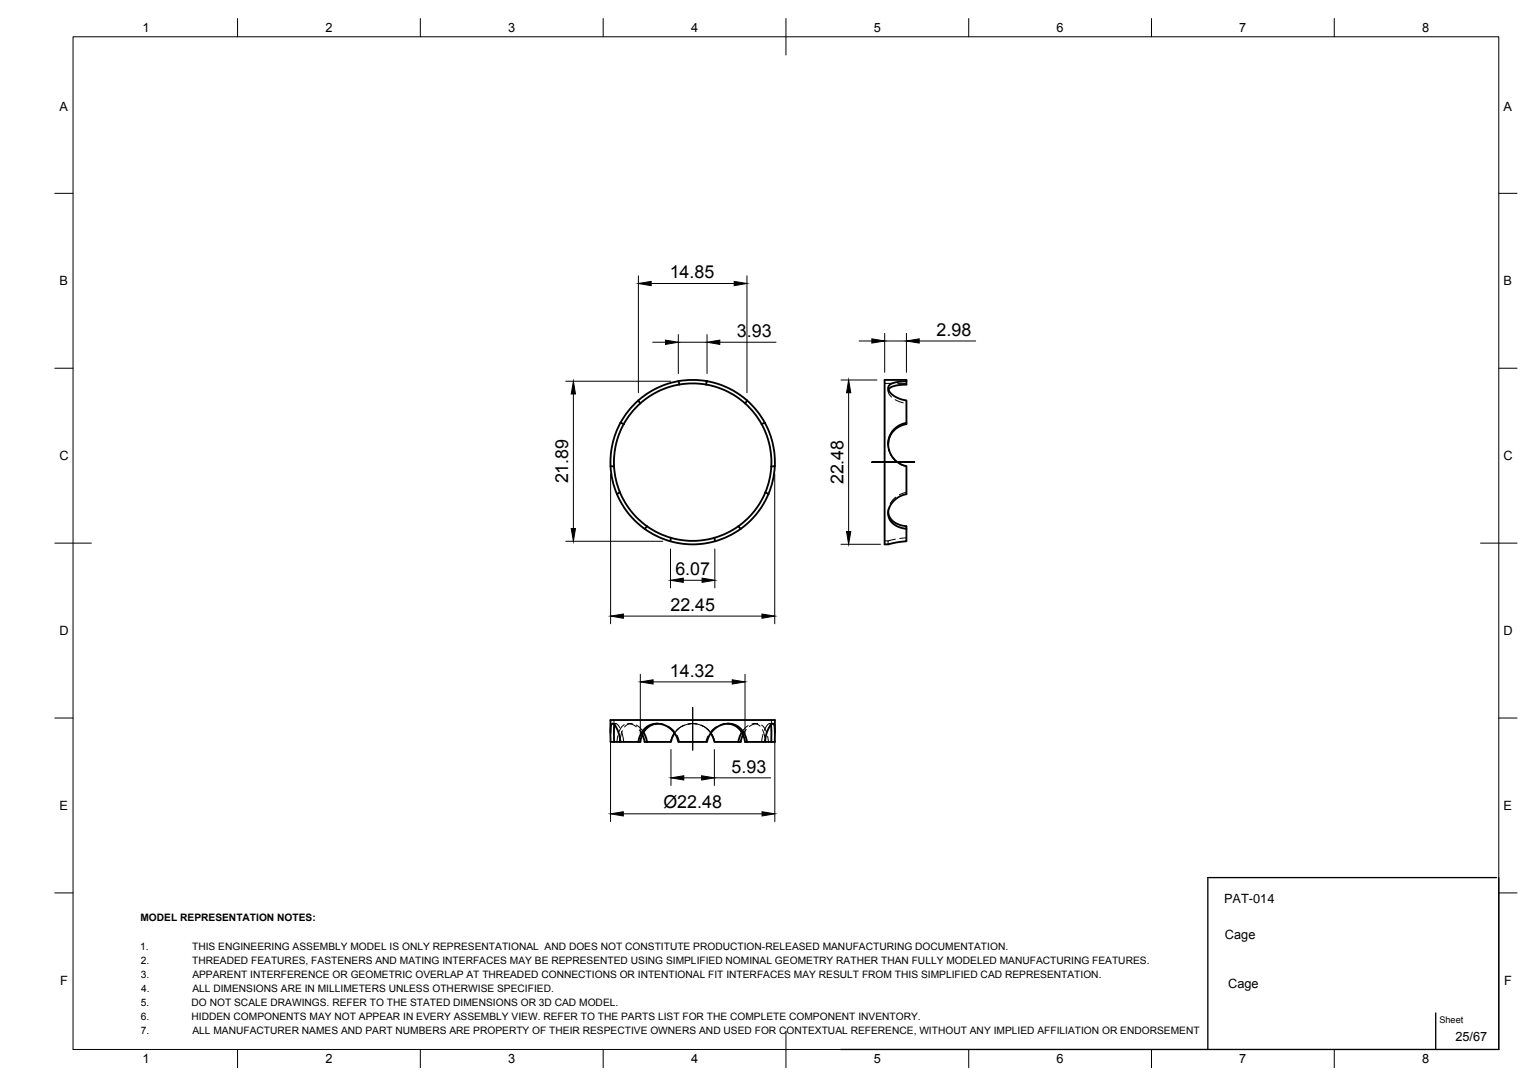
ISO-10303-21;
HEADER;
/* Generated by software containing ST-Developer
 * from STEP Tools, Inc. (www.steptools.com) 
 */

FILE_DESCRIPTION(
/* description */ ('Bin tilter linkage'),
/* implementation_level */ '2;1');

FILE_NAME(
/* name */ 'Cage.step',
/* time_stamp */ '2026-10-28T03:26:24-07:00',
/* author */ (''),
/* organization */ (''),
/* preprocessor_version */ 'ST-DEVELOPER v20.2',
/* originating_system */ 'Autodesk Translation Framework v15.17.0.0',
/* authorisation */ '');

FILE_SCHEMA (('AUTOMOTIVE_DESIGN { 1 0 10303 214 3 1 1 }'));
ENDSEC;

DATA;
#10=MECHANICAL_DESIGN_GEOMETRIC_PRESENTATION_REPRESENTATION('',(#943),#23728);
#599=B_SPLINE_CURVE_WITH_KNOTS('',3,(#21962,#21963,#21964,#21965,#21966,
#21967,#21968,#21969,#21970,#21971,#21972,#21973,#21974,#21975,#21976,#21977,
#21978,#21979,#21980,#21981,#21982,#21983),.UNSPECIFIED.,.F.,.F.,(4,2,2,
2,2,2,2,2,2,2,4),(0.0591825211272536,0.157966726598481,0.236950089897721,
0.315933453196962,0.391576304923761,0.46721915665056,0.54286200837736,0.618504860104159,
0.697488223403399,0.77647158670264,0.875255792173867),.UNSPECIFIED.);
#600=B_SPLINE_CURVE_WITH_KNOTS('',3,(#21987,#21988,#21989,#21990,#21991,
#21992,#21993,#21994,#21995,#21996,#21997,#21998,#21999,#22000,#22001,#22002,
#22003,#22004,#22005,#22006,#22007,#22008),.UNSPECIFIED.,.F.,.F.,(4,2,2,
2,2,2,2,2,2,2,4),(0.0581119756758434,0.106553146291161,0.213106292582322,
0.30849933801665,0.386091982889075,0.4636846277615,0.541277272633925,0.61886991750635,
0.714262962940678,0.820816109231839,0.869257279847157),.UNSPECIFIED.);
#601=B_SPLINE_CURVE_WITH_KNOTS('',3,(#22014,#22015,#22016,#22017,#22018,
#22019,#22020,#22021,#22022,#22023,#22024,#22025,#22026,#22027,#22028,#22029,
#22030,#22031,#22032,#22033,#22034,#22035),.UNSPECIFIED.,.F.,.F.,(4,2,2,
2,2,2,2,2,2,2,4),(0.0581119756758434,0.106553146291161,0.213106292582322,
0.30849933801665,0.386091982889075,0.4636846277615,0.541277272633925,0.61886991750635,
0.714262962940679,0.820816109231839,0.869257279847157),.UNSPECIFIED.);
#602=B_SPLINE_CURVE_WITH_KNOTS('',3,(#22039,#22040,#22041,#22042,#22043,
#22044,#22045,#22046,#22047,#22048,#22049,#22050,#22051,#22052,#22053,#22054,
#22055,#22056,#22057,#22058,#22059,#22060),.UNSPECIFIED.,.F.,.F.,(4,2,2,
2,2,2,2,2,2,2,4),(0.0581119756758433,0.106553146291161,0.213106292582322,
0.308499338016649,0.386091982889075,0.4636846277615,0.541277272633925,0.61886991750635,
0.714262962940678,0.820816109231839,0.869257279847157),.UNSPECIFIED.);
#603=B_SPLINE_CURVE_WITH_KNOTS('',3,(#22069,#22070,#22071,#22072,#22073,
#22074,#22075,#22076,#22077,#22078,#22079,#22080,#22081,#22082,#22083,#22084,
#22085,#22086,#22087,#22088,#22089,#22090),.UNSPECIFIED.,.F.,.F.,(4,2,2,
2,2,2,2,2,2,2,4),(0.0581119756758433,0.106553146291161,0.213106292582322,
0.30849933801665,0.386091982889075,0.4636846277615,0.541277272633925,0.61886991750635,
0.714262962940678,0.820816109231839,0.869257279847157),.UNSPECIFIED.);
#604=B_SPLINE_CURVE_WITH_KNOTS('',3,(#22094,#22095,#22096,#22097,#22098,
#22099,#22100,#22101,#22102,#22103,#22104,#22105,#22106,#22107,#22108,#22109,
#22110,#22111,#22112,#22113,#22114,#22115),.UNSPECIFIED.,.F.,.F.,(4,2,2,
2,2,2,2,2,2,2,4),(0.0581119756758434,0.106553146291161,0.213106292582322,
0.30849933801665,0.386091982889075,0.4636846277615,0.541277272633925,0.61886991750635,
0.714262962940678,0.820816109231839,0.869257279847157),.UNSPECIFIED.);
#605=B_SPLINE_CURVE_WITH_KNOTS('',3,(#22119,#22120,#22121,#22122,#22123,
#22124,#22125,#22126,#22127,#22128,#22129,#22130,#22131,#22132,#22133,#22134,
#22135,#22136,#22137,#22138,#22139,#22140),.UNSPECIFIED.,.F.,.F.,(4,2,2,
2,2,2,2,2,2,2,4),(0.0581119756758434,0.106553146291161,0.213106292582322,
0.30849933801665,0.386091982889075,0.4636846277615,0.541277272633925,0.61886991750635,
0.714262962940678,0.820816109231839,0.869257279847157),.UNSPECIFIED.);
#606=B_SPLINE_CURVE_WITH_KNOTS('',3,(#22144,#22145,#22146,#22147,#22148,
#22149,#22150,#22151,#22152,#22153,#22154,#22155,#22156,#22157,#22158,#22159,
#22160,#22161,#22162,#22163,#22164,#22165),.UNSPECIFIED.,.F.,.F.,(4,2,2,
2,2,2,2,2,2,2,4),(0.0581119756758433,0.106553146291161,0.213106292582322,
0.30849933801665,0.386091982889075,0.4636846277615,0.541277272633925,0.61886991750635,
0.714262962940678,0.820816109231839,0.869257279847157),.UNSPECIFIED.);
#607=B_SPLINE_CURVE_WITH_KNOTS('',3,(#22173,#22174,#22175,#22176,#22177,
#22178,#22179,#22180,#22181,#22182,#22183,#22184,#22185,#22186,#22187,#22188,
#22189,#22190,#22191,#22192,#22193,#22194),.UNSPECIFIED.,.F.,.F.,(4,2,2,
2,2,2,2,2,2,2,4),(0.0591825211272536,0.157966726598481,0.236950089897721,
0.315933453196962,0.391576304923761,0.467219156650561,0.54286200837736,
0.618504860104159,0.697488223403399,0.77647158670264,0.875255792173867),
 .UNSPECIFIED.);
#608=B_SPLINE_CURVE_WITH_KNOTS('',3,(#22202,#22203,#22204,#22205,#22206,
#22207,#22208,#22209,#22210,#22211,#22212,#22213,#22214,#22215,#22216,#22217,
#22218,#22219,#22220,#22221,#22222,#22223),.UNSPECIFIED.,.F.,.F.,(4,2,2,
2,2,2,2,2,2,2,4),(0.0591825211272536,0.157966726598481,0.236950089897722,
0.315933453196962,0.391576304923761,0.467219156650561,0.54286200837736,
0.618504860104159,0.697488223403399,0.77647158670264,0.875255792173867),
 .UNSPECIFIED.);
#609=B_SPLINE_CURVE_WITH_KNOTS('',3,(#22233,#22234,#22235,#22236,#22237,
#22238,#22239,#22240,#22241,#22242,#22243,#22244,#22245,#22246,#22247,#22248,
#22249,#22250,#22251,#22252,#22253,#22254),.UNSPECIFIED.,.F.,.F.,(4,2,2,
2,2,2,2,2,2,2,4),(0.0591825211272536,0.157966726598481,0.236950089897721,
0.315933453196962,0.391576304923761,0.46721915665056,0.54286200837736,0.618504860104159,
0.697488223403399,0.77647158670264,0.875255792173867),.UNSPECIFIED.);
#610=B_SPLINE_CURVE_WITH_KNOTS('',3,(#22262,#22263,#22264,#22265,#22266,
#22267,#22268,#22269,#22270,#22271,#22272,#22273,#22274,#22275,#22276,#22277,
#22278,#22279,#22280,#22281,#22282,#22283),.UNSPECIFIED.,.F.,.F.,(4,2,2,
2,2,2,2,2,2,2,4),(0.0591825211272536,0.157966726598481,0.236950089897721,
0.315933453196962,0.391576304923761,0.46721915665056,0.542862008377359,
0.618504860104159,0.697488223403399,0.776471586702639,0.875255792173867),
 .UNSPECIFIED.);
#611=B_SPLINE_CURVE_WITH_KNOTS('',3,(#22291,#22292,#22293,#22294,#22295,
#22296,#22297,#22298,#22299,#22300,#22301,#22302,#22303,#22304,#22305,#22306,
#22307,#22308,#22309,#22310,#22311,#22312),.UNSPECIFIED.,.F.,.F.,(4,2,2,
2,2,2,2,2,2,2,4),(0.0591825211272536,0.157966726598481,0.236950089897721,
0.315933453196962,0.391576304923761,0.46721915665056,0.54286200837736,0.618504860104159,
0.697488223403399,0.77647158670264,0.875255792173867),.UNSPECIFIED.);
#612=B_SPLINE_CURVE_WITH_KNOTS('',3,(#22321,#22322,#22323,#22324,#22325,
#22326,#22327,#22328,#22329,#22330,#22331,#22332,#22333,#22334,#22335,#22336,
#22337,#22338,#22339,#22340,#22341,#22342),.UNSPECIFIED.,.F.,.F.,(4,2,2,
2,2,2,2,2,2,2,4),(0.0591825211272536,0.157966726598481,0.236950089897721,
0.315933453196962,0.391576304923761,0.46721915665056,0.542862008377359,
0.618504860104159,0.697488223403399,0.776471586702639,0.875255792173867),
 .UNSPECIFIED.);
#620=SPHERICAL_SURFACE('',#14830,0.309556);
#621=SPHERICAL_SURFACE('',#14846,0.309556);
#622=SPHERICAL_SURFACE('',#14851,0.309556);
#623=SPHERICAL_SURFACE('',#14857,0.309556);
#624=SPHERICAL_SURFACE('',#14862,0.309556);
#625=SPHERICAL_SURFACE('',#14867,0.309556);
#626=SPHERICAL_SURFACE('',#14875,0.309556);
#725=SHAPE_REPRESENTATION_RELATIONSHIP('SRR','None',#24192,#831);
#831=ADVANCED_BREP_SHAPE_REPRESENTATION('',(#1056),#23692);
#943=STYLED_ITEM('',(#24765),#1056);
#1056=MANIFOLD_SOLID_BREP('Continuous crown cage',#12474);
#1390=FACE_BOUND('',#3514,.T.);
#1741=PLANE('',#14843);
#1742=PLANE('',#14848);
#1743=PLANE('',#14853);
#1744=PLANE('',#14859);
#1745=PLANE('',#14864);
#1746=PLANE('',#14873);
#1747=PLANE('',#14877);
#1748=PLANE('',#14878);
#2418=FACE_OUTER_BOUND('',#3498,.T.);
#2419=FACE_OUTER_BOUND('',#3499,.T.);
#2420=FACE_OUTER_BOUND('',#3500,.T.);
#2421=FACE_OUTER_BOUND('',#3501,.T.);
#2422=FACE_OUTER_BOUND('',#3502,.T.);
#2423=FACE_OUTER_BOUND('',#3503,.T.);
#2424=FACE_OUTER_BOUND('',#3504,.T.);
#2425=FACE_OUTER_BOUND('',#3505,.T.);
#2426=FACE_OUTER_BOUND('',#3506,.T.);
#2427=FACE_OUTER_BOUND('',#3507,.T.);
#2428=FACE_OUTER_BOUND('',#3508,.T.);
#2429=FACE_OUTER_BOUND('',#3509,.T.);
#2430=FACE_OUTER_BOUND('',#3510,.T.);
#2431=FACE_OUTER_BOUND('',#3511,.T.);
#2432=FACE_OUTER_BOUND('',#3512,.T.);
#2433=FACE_OUTER_BOUND('',#3513,.T.);
#2434=FACE_OUTER_BOUND('',#3515,.T.);
#3498=EDGE_LOOP('',(#10291,#10292,#10293,#10294));
#3499=EDGE_LOOP('',(#10295,#10296,#10297,#10298,#10299,#10300,#10301,#10302,
#10303,#10304,#10305,#10306,#10307,#10308,#10309,#10310,#10311,#10312));
#3500=EDGE_LOOP('',(#10313,#10314,#10315,#10316));
#3501=EDGE_LOOP('',(#10317,#10318,#10319,#10320));
#3502=EDGE_LOOP('',(#10321,#10322,#10323,#10324));
#3503=EDGE_LOOP('',(#10325,#10326,#10327,#10328));
#3504=EDGE_LOOP('',(#10329,#10330,#10331,#10332,#10333,#10334));
#3505=EDGE_LOOP('',(#10335,#10336,#10337,#10338));
#3506=EDGE_LOOP('',(#10339,#10340,#10341,#10342));
#3507=EDGE_LOOP('',(#10343,#10344,#10345,#10346));
#3508=EDGE_LOOP('',(#10347,#10348,#10349,#10350));
#3509=EDGE_LOOP('',(#10351,#10352,#10353,#10354));
#3510=EDGE_LOOP('',(#10355,#10356,#10357,#10358,#10359,#10360,#10361,#10362,
#10363,#10364,#10365,#10366,#10367,#10368,#10369,#10370,#10371,#10372));
#3511=EDGE_LOOP('',(#10373,#10374,#10375,#10376));
#3512=EDGE_LOOP('',(#10377,#10378,#10379,#10380));
#3513=EDGE_LOOP('',(#10381));
#3514=EDGE_LOOP('',(#10382));
#3515=EDGE_LOOP('',(#10383,#10384,#10385,#10386));
#4263=LINE('',#22064,#4938);
#4264=LINE('',#22317,#4939);
#4938=VECTOR('',#18210,1.123812);
#4939=VECTOR('',#18279,1.076188);
#5744=CIRCLE('',#14831,0.303778037777585);
#5745=CIRCLE('',#14832,0.303778037777585);
#5746=CIRCLE('',#14834,1.123812);
#5747=CIRCLE('',#14835,1.123812);
#5748=CIRCLE('',#14836,1.123812);
#5749=CIRCLE('',#14837,1.123812);
#5750=CIRCLE('',#14838,1.123812);
#5751=CIRCLE('',#14839,1.123812);
#5752=CIRCLE('',#14840,1.123812);
#5753=CIRCLE('',#14841,1.123812);
#5754=CIRCLE('',#14842,1.123812);
#5755=CIRCLE('',#14844,1.076188);
#5756=CIRCLE('',#14845,0.303778037777585);
#5757=CIRCLE('',#14847,0.303778037777585);
#5758=CIRCLE('',#14849,1.076188);
#5759=CIRCLE('',#14850,0.303778037777585);
#5760=CIRCLE('',#14852,0.303778037777585);
#5761=CIRCLE('',#14854,1.076188);
#5762=CIRCLE('',#14855,1.076188);
#5763=CIRCLE('',#14856,0.303778037777585);
#5764=CIRCLE('',#14858,0.303778037777585);
#5765=CIRCLE('',#14860,1.076188);
#5766=CIRCLE('',#14861,0.303778037777585);
#5767=CIRCLE('',#14863,0.303778037777585);
#5768=CIRCLE('',#14865,1.076188);
#5769=CIRCLE('',#14866,0.303778037777585);
#5770=CIRCLE('',#14868,0.303778037777585);
#5771=CIRCLE('',#14870,1.076188);
#5772=CIRCLE('',#14871,1.076188);
#5773=CIRCLE('',#14872,1.076188);
#5774=CIRCLE('',#14874,0.303778037777585);
#5775=CIRCLE('',#14876,0.303778037777585);
#6603=VERTEX_POINT('',#21960);
#6604=VERTEX_POINT('',#21961);
#6605=VERTEX_POINT('',#21984);
#6606=VERTEX_POINT('',#21986);
#6607=VERTEX_POINT('',#22011);
#6608=VERTEX_POINT('',#22013);
#6609=VERTEX_POINT('',#22036);
#6610=VERTEX_POINT('',#22038);
#6611=VERTEX_POINT('',#22061);
#6612=VERTEX_POINT('',#22063);
#6613=VERTEX_POINT('',#22066);
#6614=VERTEX_POINT('',#22068);
#6615=VERTEX_POINT('',#22091);
#6616=VERTEX_POINT('',#22093);
#6617=VERTEX_POINT('',#22116);
#6618=VERTEX_POINT('',#22118);
#6619=VERTEX_POINT('',#22141);
#6620=VERTEX_POINT('',#22143);
#6621=VERTEX_POINT('',#22168);
#6622=VERTEX_POINT('',#22172);
#6623=VERTEX_POINT('',#22197);
#6624=VERTEX_POINT('',#22201);
#6625=VERTEX_POINT('',#22226);
#6626=VERTEX_POINT('',#22228);
#6627=VERTEX_POINT('',#22232);
#6628=VERTEX_POINT('',#22257);
#6629=VERTEX_POINT('',#22261);
#6630=VERTEX_POINT('',#22286);
#6631=VERTEX_POINT('',#22290);
#6632=VERTEX_POINT('',#22315);
#6633=VERTEX_POINT('',#22318);
#6634=VERTEX_POINT('',#22320);
#7885=EDGE_CURVE('',#6603,#6604,#599,.T.);
#7886=EDGE_CURVE('',#6605,#6603,#5744,.T.);
#7887=EDGE_CURVE('',#6606,#6605,#600,.T.);
#7888=EDGE_CURVE('',#6604,#6606,#5745,.T.);
#7889=EDGE_CURVE('',#6607,#6605,#5746,.T.);
#7890=EDGE_CURVE('',#6607,#6608,#601,.T.);
#7891=EDGE_CURVE('',#6609,#6608,#5747,.T.);
#7892=EDGE_CURVE('',#6609,#6610,#602,.T.);
#7893=EDGE_CURVE('',#6611,#6610,#5748,.T.);
#7894=EDGE_CURVE('',#6611,#6612,#4263,.T.);
#7895=EDGE_CURVE('',#6612,#6612,#5749,.T.);
#7896=EDGE_CURVE('',#6613,#6611,#5750,.T.);
#7897=EDGE_CURVE('',#6613,#6614,#603,.T.);
#7898=EDGE_CURVE('',#6615,#6614,#5751,.T.);
#7899=EDGE_CURVE('',#6615,#6616,#604,.T.);
#7900=EDGE_CURVE('',#6617,#6616,#5752,.T.);
#7901=EDGE_CURVE('',#6617,#6618,#605,.T.);
#7902=EDGE_CURVE('',#6619,#6618,#5753,.T.);
#7903=EDGE_CURVE('',#6619,#6620,#606,.T.);
#7904=EDGE_CURVE('',#6606,#6620,#5754,.T.);
#7905=EDGE_CURVE('',#6603,#6621,#5755,.T.);
#7906=EDGE_CURVE('',#6621,#6607,#5756,.T.);
#7907=EDGE_CURVE('',#6622,#6621,#607,.T.);
#7908=EDGE_CURVE('',#6608,#6622,#5757,.T.);
#7909=EDGE_CURVE('',#6622,#6623,#5758,.T.);
#7910=EDGE_CURVE('',#6623,#6609,#5759,.T.);
#7911=EDGE_CURVE('',#6624,#6623,#608,.T.);
#7912=EDGE_CURVE('',#6610,#6624,#5760,.T.);
#7913=EDGE_CURVE('',#6624,#6625,#5761,.T.);
#7914=EDGE_CURVE('',#6625,#6626,#5762,.T.);
#7915=EDGE_CURVE('',#6626,#6613,#5763,.T.);
#7916=EDGE_CURVE('',#6627,#6626,#609,.T.);
#7917=EDGE_CURVE('',#6614,#6627,#5764,.T.);
#7918=EDGE_CURVE('',#6627,#6628,#5765,.T.);
#7919=EDGE_CURVE('',#6628,#6615,#5766,.T.);
#7920=EDGE_CURVE('',#6629,#6628,#610,.T.);
#7921=EDGE_CURVE('',#6616,#6629,#5767,.T.);
#7922=EDGE_CURVE('',#6629,#6630,#5768,.T.);
#7923=EDGE_CURVE('',#6630,#6617,#5769,.T.);
#7924=EDGE_CURVE('',#6631,#6630,#611,.T.);
#7925=EDGE_CURVE('',#6618,#6631,#5770,.T.);
#7926=EDGE_CURVE('',#6632,#6632,#5771,.T.);
#7927=EDGE_CURVE('',#6632,#6625,#4264,.T.);
#7928=EDGE_CURVE('',#6633,#6604,#5772,.T.);
#7929=EDGE_CURVE('',#6633,#6634,#612,.T.);
#7930=EDGE_CURVE('',#6631,#6634,#5773,.T.);
#7931=EDGE_CURVE('',#6620,#6633,#5774,.T.);
#7932=EDGE_CURVE('',#6634,#6619,#5775,.T.);
#10291=ORIENTED_EDGE('',*,*,#7885,.F.);
#10292=ORIENTED_EDGE('',*,*,#7886,.F.);
#10293=ORIENTED_EDGE('',*,*,#7887,.F.);
#10294=ORIENTED_EDGE('',*,*,#7888,.F.);
#10295=ORIENTED_EDGE('',*,*,#7887,.T.);
#10296=ORIENTED_EDGE('',*,*,#7889,.F.);
#10297=ORIENTED_EDGE('',*,*,#7890,.T.);
#10298=ORIENTED_EDGE('',*,*,#7891,.F.);
#10299=ORIENTED_EDGE('',*,*,#7892,.T.);
#10300=ORIENTED_EDGE('',*,*,#7893,.F.);
#10301=ORIENTED_EDGE('',*,*,#7894,.T.);
#10302=ORIENTED_EDGE('',*,*,#7895,.F.);
#10303=ORIENTED_EDGE('',*,*,#7894,.F.);
#10304=ORIENTED_EDGE('',*,*,#7896,.F.);
#10305=ORIENTED_EDGE('',*,*,#7897,.T.);
#10306=ORIENTED_EDGE('',*,*,#7898,.F.);
#10307=ORIENTED_EDGE('',*,*,#7899,.T.);
#10308=ORIENTED_EDGE('',*,*,#7900,.F.);
#10309=ORIENTED_EDGE('',*,*,#7901,.T.);
#10310=ORIENTED_EDGE('',*,*,#7902,.F.);
#10311=ORIENTED_EDGE('',*,*,#7903,.T.);
#10312=ORIENTED_EDGE('',*,*,#7904,.F.);
#10313=ORIENTED_EDGE('',*,*,#7886,.T.);
#10314=ORIENTED_EDGE('',*,*,#7905,.T.);
#10315=ORIENTED_EDGE('',*,*,#7906,.T.);
#10316=ORIENTED_EDGE('',*,*,#7889,.T.);
#10317=ORIENTED_EDGE('',*,*,#7907,.F.);
#10318=ORIENTED_EDGE('',*,*,#7908,.F.);
#10319=ORIENTED_EDGE('',*,*,#7890,.F.);
#10320=ORIENTED_EDGE('',*,*,#7906,.F.);
#10321=ORIENTED_EDGE('',*,*,#7908,.T.);
#10322=ORIENTED_EDGE('',*,*,#7909,.T.);
#10323=ORIENTED_EDGE('',*,*,#7910,.T.);
#10324=ORIENTED_EDGE('',*,*,#7891,.T.);
#10325=ORIENTED_EDGE('',*,*,#7911,.F.);
#10326=ORIENTED_EDGE('',*,*,#7912,.F.);
#10327=ORIENTED_EDGE('',*,*,#7892,.F.);
#10328=ORIENTED_EDGE('',*,*,#7910,.F.);
#10329=ORIENTED_EDGE('',*,*,#7912,.T.);
#10330=ORIENTED_EDGE('',*,*,#7913,.T.);
#10331=ORIENTED_EDGE('',*,*,#7914,.T.);
#10332=ORIENTED_EDGE('',*,*,#7915,.T.);
#10333=ORIENTED_EDGE('',*,*,#7896,.T.);
#10334=ORIENTED_EDGE('',*,*,#7893,.T.);
#10335=ORIENTED_EDGE('',*,*,#7916,.F.);
#10336=ORIENTED_EDGE('',*,*,#7917,.F.);
#10337=ORIENTED_EDGE('',*,*,#7897,.F.);
#10338=ORIENTED_EDGE('',*,*,#7915,.F.);
#10339=ORIENTED_EDGE('',*,*,#7917,.T.);
#10340=ORIENTED_EDGE('',*,*,#7918,.T.);
#10341=ORIENTED_EDGE('',*,*,#7919,.T.);
#10342=ORIENTED_EDGE('',*,*,#7898,.T.);
#10343=ORIENTED_EDGE('',*,*,#7920,.F.);
#10344=ORIENTED_EDGE('',*,*,#7921,.F.);
#10345=ORIENTED_EDGE('',*,*,#7899,.F.);
#10346=ORIENTED_EDGE('',*,*,#7919,.F.);
#10347=ORIENTED_EDGE('',*,*,#7921,.T.);
#10348=ORIENTED_EDGE('',*,*,#7922,.T.);
#10349=ORIENTED_EDGE('',*,*,#7923,.T.);
#10350=ORIENTED_EDGE('',*,*,#7900,.T.);
#10351=ORIENTED_EDGE('',*,*,#7901,.F.);
#10352=ORIENTED_EDGE('',*,*,#7923,.F.);
#10353=ORIENTED_EDGE('',*,*,#7924,.F.);
#10354=ORIENTED_EDGE('',*,*,#7925,.F.);
#10355=ORIENTED_EDGE('',*,*,#7926,.F.);
#10356=ORIENTED_EDGE('',*,*,#7927,.T.);
#10357=ORIENTED_EDGE('',*,*,#7913,.F.);
#10358=ORIENTED_EDGE('',*,*,#7911,.T.);
#10359=ORIENTED_EDGE('',*,*,#7909,.F.);
#10360=ORIENTED_EDGE('',*,*,#7907,.T.);
#10361=ORIENTED_EDGE('',*,*,#7905,.F.);
#10362=ORIENTED_EDGE('',*,*,#7885,.T.);
#10363=ORIENTED_EDGE('',*,*,#7928,.F.);
#10364=ORIENTED_EDGE('',*,*,#7929,.T.);
#10365=ORIENTED_EDGE('',*,*,#7930,.F.);
#10366=ORIENTED_EDGE('',*,*,#7924,.T.);
#10367=ORIENTED_EDGE('',*,*,#7922,.F.);
#10368=ORIENTED_EDGE('',*,*,#7920,.T.);
#10369=ORIENTED_EDGE('',*,*,#7918,.F.);
#10370=ORIENTED_EDGE('',*,*,#7916,.T.);
#10371=ORIENTED_EDGE('',*,*,#7914,.F.);
#10372=ORIENTED_EDGE('',*,*,#7927,.F.);
#10373=ORIENTED_EDGE('',*,*,#7888,.T.);
#10374=ORIENTED_EDGE('',*,*,#7904,.T.);
#10375=ORIENTED_EDGE('',*,*,#7931,.T.);
#10376=ORIENTED_EDGE('',*,*,#7928,.T.);
#10377=ORIENTED_EDGE('',*,*,#7903,.F.);
#10378=ORIENTED_EDGE('',*,*,#7932,.F.);
#10379=ORIENTED_EDGE('',*,*,#7929,.F.);
#10380=ORIENTED_EDGE('',*,*,#7931,.F.);
#10381=ORIENTED_EDGE('',*,*,#7895,.T.);
#10382=ORIENTED_EDGE('',*,*,#7926,.T.);
#10383=ORIENTED_EDGE('',*,*,#7925,.T.);
#10384=ORIENTED_EDGE('',*,*,#7930,.T.);
#10385=ORIENTED_EDGE('',*,*,#7932,.T.);
#10386=ORIENTED_EDGE('',*,*,#7902,.T.);
#11529=CYLINDRICAL_SURFACE('',#14833,1.123812);
#11530=CYLINDRICAL_SURFACE('',#14869,1.076188);
#12143=ADVANCED_FACE('',(#2418),#620,.F.);
#12144=ADVANCED_FACE('',(#2419),#11529,.T.);
#12145=ADVANCED_FACE('',(#2420),#1741,.T.);
#12146=ADVANCED_FACE('',(#2421),#621,.F.);
#12147=ADVANCED_FACE('',(#2422),#1742,.T.);
#12148=ADVANCED_FACE('',(#2423),#622,.F.);
#12149=ADVANCED_FACE('',(#2424),#1743,.T.);
#12150=ADVANCED_FACE('',(#2425),#623,.F.);
#12151=ADVANCED_FACE('',(#2426),#1744,.T.);
#12152=ADVANCED_FACE('',(#2427),#624,.F.);
#12153=ADVANCED_FACE('',(#2428),#1745,.T.);
#12154=ADVANCED_FACE('',(#2429),#625,.F.);
#12155=ADVANCED_FACE('',(#2430),#11530,.F.);
#12156=ADVANCED_FACE('',(#2431),#1746,.T.);
#12157=ADVANCED_FACE('',(#2432),#626,.F.);
#12158=ADVANCED_FACE('',(#2433,#1390),#1747,.T.);
#12159=ADVANCED_FACE('',(#2434),#1748,.T.);
#12474=CLOSED_SHELL('',(#12143,#12144,#12145,#12146,#12147,#12148,#12149,
#12150,#12151,#12152,#12153,#12154,#12155,#12156,#12157,#12158,#12159));
#14829=AXIS2_PLACEMENT_3D('',#21958,#18194,#18195);
#14830=AXIS2_PLACEMENT_3D('',#21959,#18196,#18197);
#14831=AXIS2_PLACEMENT_3D('',#21985,#18198,#18199);
#14832=AXIS2_PLACEMENT_3D('',#22009,#18200,#18201);
#14833=AXIS2_PLACEMENT_3D('',#22010,#18202,#18203);
#14834=AXIS2_PLACEMENT_3D('',#22012,#18204,#18205);
#14835=AXIS2_PLACEMENT_3D('',#22037,#18206,#18207);
#14836=AXIS2_PLACEMENT_3D('',#22062,#18208,#18209);
#14837=AXIS2_PLACEMENT_3D('',#22065,#18211,#18212);
#14838=AXIS2_PLACEMENT_3D('',#22067,#18213,#18214);
#14839=AXIS2_PLACEMENT_3D('',#22092,#18215,#18216);
#14840=AXIS2_PLACEMENT_3D('',#22117,#18217,#18218);
#14841=AXIS2_PLACEMENT_3D('',#22142,#18219,#18220);
#14842=AXIS2_PLACEMENT_3D('',#22166,#18221,#18222);
#14843=AXIS2_PLACEMENT_3D('',#22167,#18223,#18224);
#14844=AXIS2_PLACEMENT_3D('',#22169,#18225,#18226);
#14845=AXIS2_PLACEMENT_3D('',#22170,#18227,#18228);
#14846=AXIS2_PLACEMENT_3D('',#22171,#18229,#18230);
#14847=AXIS2_PLACEMENT_3D('',#22195,#18231,#18232);
#14848=AXIS2_PLACEMENT_3D('',#22196,#18233,#18234);
#14849=AXIS2_PLACEMENT_3D('',#22198,#18235,#18236);
#14850=AXIS2_PLACEMENT_3D('',#22199,#18237,#18238);
#14851=AXIS2_PLACEMENT_3D('',#22200,#18239,#18240);
#14852=AXIS2_PLACEMENT_3D('',#22224,#18241,#18242);
#14853=AXIS2_PLACEMENT_3D('',#22225,#18243,#18244);
#14854=AXIS2_PLACEMENT_3D('',#22227,#18245,#18246);
#14855=AXIS2_PLACEMENT_3D('',#22229,#18247,#18248);
#14856=AXIS2_PLACEMENT_3D('',#22230,#18249,#18250);
#14857=AXIS2_PLACEMENT_3D('',#22231,#18251,#18252);
#14858=AXIS2_PLACEMENT_3D('',#22255,#18253,#18254);
#14859=AXIS2_PLACEMENT_3D('',#22256,#18255,#18256);
#14860=AXIS2_PLACEMENT_3D('',#22258,#18257,#18258);
#14861=AXIS2_PLACEMENT_3D('',#22259,#18259,#18260);
#14862=AXIS2_PLACEMENT_3D('',#22260,#18261,#18262);
#14863=AXIS2_PLACEMENT_3D('',#22284,#18263,#18264);
#14864=AXIS2_PLACEMENT_3D('',#22285,#18265,#18266);
#14865=AXIS2_PLACEMENT_3D('',#22287,#18267,#18268);
#14866=AXIS2_PLACEMENT_3D('',#22288,#18269,#18270);
#14867=AXIS2_PLACEMENT_3D('',#22289,#18271,#18272);
#14868=AXIS2_PLACEMENT_3D('',#22313,#18273,#18274);
#14869=AXIS2_PLACEMENT_3D('',#22314,#18275,#18276);
#14870=AXIS2_PLACEMENT_3D('',#22316,#18277,#18278);
#14871=AXIS2_PLACEMENT_3D('',#22319,#18280,#18281);
#14872=AXIS2_PLACEMENT_3D('',#22343,#18282,#18283);
#14873=AXIS2_PLACEMENT_3D('',#22344,#18284,#18285);
#14874=AXIS2_PLACEMENT_3D('',#22345,#18286,#18287);
#14875=AXIS2_PLACEMENT_3D('',#22346,#18288,#18289);
#14876=AXIS2_PLACEMENT_3D('',#22347,#18290,#18291);
#14877=AXIS2_PLACEMENT_3D('',#22348,#18292,#18293);
#14878=AXIS2_PLACEMENT_3D('',#22349,#18294,#18295);
#18194=DIRECTION('axis',(0.,0.,1.));
#18195=DIRECTION('refdir',(1.,0.,0.));
#18196=DIRECTION('center_axis',(0.,0.,1.));
#18197=DIRECTION('ref_axis',(1.,0.,0.));
#18198=DIRECTION('center_axis',(0.,-1.,0.));
#18199=DIRECTION('ref_axis',(0.,0.,-1.));
#18200=DIRECTION('center_axis',(0.,-1.,0.));
#18201=DIRECTION('ref_axis',(0.,0.,-1.));
#18202=DIRECTION('center_axis',(0.,1.,0.));
#18203=DIRECTION('ref_axis',(1.,0.,0.));
#18204=DIRECTION('center_axis',(0.,1.,0.));
#18205=DIRECTION('ref_axis',(1.,0.,0.));
#18206=DIRECTION('center_axis',(0.,1.,0.));
#18207=DIRECTION('ref_axis',(1.,0.,0.));
#18208=DIRECTION('center_axis',(0.,1.,0.));
#18209=DIRECTION('ref_axis',(1.,0.,0.));
#18210=DIRECTION('',(0.,-1.,0.));
#18211=DIRECTION('center_axis',(0.,-1.,0.));
#18212=DIRECTION('ref_axis',(1.,0.,0.));
#18213=DIRECTION('center_axis',(0.,1.,0.));
#18214=DIRECTION('ref_axis',(1.,0.,0.));
#18215=DIRECTION('center_axis',(0.,1.,0.));
#18216=DIRECTION('ref_axis',(1.,0.,0.));
#18217=DIRECTION('center_axis',(0.,1.,0.));
#18218=DIRECTION('ref_axis',(1.,0.,0.));
#18219=DIRECTION('center_axis',(0.,1.,0.));
#18220=DIRECTION('ref_axis',(1.,0.,0.));
#18221=DIRECTION('center_axis',(0.,1.,0.));
#18222=DIRECTION('ref_axis',(1.,0.,0.));
#18223=DIRECTION('center_axis',(0.,1.,0.));
#18224=DIRECTION('ref_axis',(1.,0.,0.));
#18225=DIRECTION('center_axis',(0.,-1.,0.));
#18226=DIRECTION('ref_axis',(1.,0.,0.));
#18227=DIRECTION('center_axis',(0.,-1.,0.));
#18228=DIRECTION('ref_axis',(0.,0.,-1.));
#18229=DIRECTION('center_axis',(8.96625347776458E-17,0.,1.));
#18230=DIRECTION('ref_axis',(1.,0.,0.));
#18231=DIRECTION('center_axis',(0.,-1.,0.));
#18232=DIRECTION('ref_axis',(0.,0.,-1.));
#18233=DIRECTION('center_axis',(0.,1.,0.));
#18234=DIRECTION('ref_axis',(1.,0.,0.));
#18235=DIRECTION('center_axis',(0.,-1.,0.));
#18236=DIRECTION('ref_axis',(1.,0.,0.));
#18237=DIRECTION('center_axis',(0.,-1.,0.));
#18238=DIRECTION('ref_axis',(0.,0.,-1.));
#18239=DIRECTION('center_axis',(0.,0.,1.));
#18240=DIRECTION('ref_axis',(1.,0.,0.));
#18241=DIRECTION('center_axis',(0.,-1.,0.));
#18242=DIRECTION('ref_axis',(0.,0.,-1.));
#18243=DIRECTION('center_axis',(0.,1.,0.));
#18244=DIRECTION('ref_axis',(1.,0.,0.));
#18245=DIRECTION('center_axis',(0.,-1.,0.));
#18246=DIRECTION('ref_axis',(1.,0.,0.));
#18247=DIRECTION('center_axis',(0.,-1.,0.));
#18248=DIRECTION('ref_axis',(1.,0.,0.));
#18249=DIRECTION('center_axis',(0.,-1.,0.));
#18250=DIRECTION('ref_axis',(0.,0.,-1.));
#18251=DIRECTION('center_axis',(0.,0.,1.));
#18252=DIRECTION('ref_axis',(1.,0.,0.));
#18253=DIRECTION('center_axis',(0.,-1.,0.));
#18254=DIRECTION('ref_axis',(0.,0.,-1.));
#18255=DIRECTION('center_axis',(0.,1.,0.));
#18256=DIRECTION('ref_axis',(1.,0.,0.));
#18257=DIRECTION('center_axis',(0.,-1.,0.));
#18258=DIRECTION('ref_axis',(1.,0.,0.));
#18259=DIRECTION('center_axis',(0.,-1.,0.));
#18260=DIRECTION('ref_axis',(0.,0.,-1.));
#18261=DIRECTION('center_axis',(8.96625347776458E-17,0.,1.));
#18262=DIRECTION('ref_axis',(1.,0.,0.));
#18263=DIRECTION('center_axis',(0.,-1.,0.));
#18264=DIRECTION('ref_axis',(0.,0.,-1.));
#18265=DIRECTION('center_axis',(0.,1.,0.));
#18266=DIRECTION('ref_axis',(1.,0.,0.));
#18267=DIRECTION('center_axis',(0.,-1.,0.));
#18268=DIRECTION('ref_axis',(1.,0.,0.));
#18269=DIRECTION('center_axis',(0.,-1.,0.));
#18270=DIRECTION('ref_axis',(0.,0.,-1.));
#18271=DIRECTION('center_axis',(0.,0.,1.));
#18272=DIRECTION('ref_axis',(1.,0.,0.));
#18273=DIRECTION('center_axis',(0.,-1.,0.));
#18274=DIRECTION('ref_axis',(0.,0.,-1.));
#18275=DIRECTION('center_axis',(0.,1.,0.));
#18276=DIRECTION('ref_axis',(1.,0.,0.));
#18277=DIRECTION('center_axis',(0.,1.,0.));
#18278=DIRECTION('ref_axis',(1.,0.,0.));
#18279=DIRECTION('',(0.,1.,0.));
#18280=DIRECTION('center_axis',(0.,-1.,0.));
#18281=DIRECTION('ref_axis',(1.,0.,0.));
#18282=DIRECTION('center_axis',(0.,-1.,0.));
#18283=DIRECTION('ref_axis',(1.,0.,0.));
#18284=DIRECTION('center_axis',(0.,1.,0.));
#18285=DIRECTION('ref_axis',(1.,0.,0.));
#18286=DIRECTION('center_axis',(0.,-1.,0.));
#18287=DIRECTION('ref_axis',(0.,0.,-1.));
#18288=DIRECTION('center_axis',(0.,0.,1.));
#18289=DIRECTION('ref_axis',(1.,0.,0.));
#18290=DIRECTION('center_axis',(0.,-1.,0.));
#18291=DIRECTION('ref_axis',(0.,0.,-1.));
#18292=DIRECTION('center_axis',(0.,-1.,0.));
#18293=DIRECTION('ref_axis',(-1.,0.,0.));
#18294=DIRECTION('center_axis',(0.,1.,0.));
#18295=DIRECTION('ref_axis',(1.,0.,0.));
#21958=CARTESIAN_POINT('',(0.,0.,0.));
#21959=CARTESIAN_POINT('Origin',(0.685838782044607,0.,0.860014630714833));
#21960=CARTESIAN_POINT('',(0.413083465285518,-0.05953,0.993751811093549));
#21961=CARTESIAN_POINT('',(0.876916659919095,-0.05953,0.623857181492959));
#21962=CARTESIAN_POINT('Ctrl Pts',(0.413083465285518,-0.05953,0.993751811093549));
#21963=CARTESIAN_POINT('Ctrl Pts',(0.419070565453383,-0.0925528133349865,
0.991263089003441));
#21964=CARTESIAN_POINT('Ctrl Pts',(0.430199341854858,-0.124911173756694,
0.986608710139579));
#21965=CARTESIAN_POINT('Ctrl Pts',(0.457978755888596,-0.177924977804098,
0.973971221090534));
#21966=CARTESIAN_POINT('Ctrl Pts',(0.473077587363685,-0.199697230012983,
0.966820759530997));
#21967=CARTESIAN_POINT('Ctrl Pts',(0.507057380724533,-0.237895043532788,
0.949440676105255));
#21968=CARTESIAN_POINT('Ctrl Pts',(0.525933334162555,-0.254319232363049,
0.939198248544428));
#21969=CARTESIAN_POINT('Ctrl Pts',(0.564362943424238,-0.28018331644634,
0.916597376014514));
#21970=CARTESIAN_POINT('Ctrl Pts',(0.585840553788742,-0.29104845371857,
0.903141581680914));
#21971=CARTESIAN_POINT('Ctrl Pts',(0.629305439856167,-0.30527573347708,
0.873412008702649));
#21972=CARTESIAN_POINT('Ctrl Pts',(0.651278921914856,-0.308638795020976,
0.857118508332695));
#21973=CARTESIAN_POINT('Ctrl Pts',(0.690705563850638,-0.308638795020976,
0.825676810575914));
#21974=CARTESIAN_POINT('Ctrl Pts',(0.711480111898423,-0.30527573347708,
0.807879894508811));
#21975=CARTESIAN_POINT('Ctrl Pts',(0.750136149454208,-0.29104845371857,
0.772120216227122));
#21976=CARTESIAN_POINT('Ctrl Pts',(0.768033796848072,-0.28018331644634,
0.754175290318038));
#21977=CARTESIAN_POINT('Ctrl Pts',(0.798619410861634,-0.254319232363049,
0.721738358858166));
#21978=CARTESIAN_POINT('Ctrl Pts',(0.812805334167529,-0.237895043532788,
0.705614819529209));
#21979=CARTESIAN_POINT('Ctrl Pts',(0.837310877969633,-0.199697230012983,
0.676354402927683));
#21980=CARTESIAN_POINT('Ctrl Pts',(0.847641868610495,-0.177924977804098,
0.663225258065736));
#21981=CARTESIAN_POINT('Ctrl Pts',(0.866144010579847,-0.124911173756694,
0.638954437806245));
#21982=CARTESIAN_POINT('Ctrl Pts',(0.873158080166742,-0.0925528133349865,
0.62914037979579));
#21983=CARTESIAN_POINT('Ctrl Pts',(0.876916659919095,-0.05953,0.623857181492959));
#21984=CARTESIAN_POINT('',(0.437601487681057,-0.05953,1.03511272300331));
#21985=CARTESIAN_POINT('Origin',(0.685838782044607,-0.05953,0.860014630714833));
#21986=CARTESIAN_POINT('',(0.911784794170997,-0.05953,0.656964154625313));
#21987=CARTESIAN_POINT('Ctrl Pts',(0.911784794170998,-0.0595300000000001,
0.656964154625312));
#21988=CARTESIAN_POINT('Ctrl Pts',(0.909827729890942,-0.0762225747374255,
0.659680317203144));
#21989=CARTESIAN_POINT('Ctrl Pts',(0.907004864562642,-0.0928409665394228,
0.663576540841106));
#21990=CARTESIAN_POINT('Ctrl Pts',(0.895234408667242,-0.144299303100741,
0.679480524217551));
#21991=CARTESIAN_POINT('Ctrl Pts',(0.882797231409153,-0.177024326825049,
0.695831250979106));
#21992=CARTESIAN_POINT('Ctrl Pts',(0.854332839576145,-0.227269801620064,
0.73042219438957));
#21993=CARTESIAN_POINT('Ctrl Pts',(0.834863020612702,-0.251265615809407,
0.752807465209441));
#21994=CARTESIAN_POINT('Ctrl Pts',(0.800439809856111,-0.279889827963178,
0.789147407129766));
#21995=CARTESIAN_POINT('Ctrl Pts',(0.781998747691871,-0.290879136862659,
0.80756613568454));
#21996=CARTESIAN_POINT('Ctrl Pts',(0.742239891936898,-0.305251990234487,
0.844254137480382));
#21997=CARTESIAN_POINT('Ctrl Pts',(0.720906778729541,-0.308638795020976,
0.862505527716294));
#21998=CARTESIAN_POINT('Ctrl Pts',(0.680463863683392,-0.308638795020976,
0.894757676234429));
#21999=CARTESIAN_POINT('Ctrl Pts',(0.657923009631182,-0.305251990234488,
0.91149460735272));
#22000=CARTESIAN_POINT('Ctrl Pts',(0.613307674922609,-0.290879136862659,
0.942092777160053));
#22001=CARTESIAN_POINT('Ctrl Pts',(0.591247219971725,-0.279889827963178,
0.955972930713954));
#22002=CARTESIAN_POINT('Ctrl Pts',(0.548158511259202,-0.251265615809407,
0.981446681891443));
#22003=CARTESIAN_POINT('Ctrl Pts',(0.522002043615455,-0.227269801620063,
0.995447160474328));
#22004=CARTESIAN_POINT('Ctrl Pts',(0.481944444320713,-0.177024326825049,
1.01550068154148));
#22005=CARTESIAN_POINT('Ctrl Pts',(0.463236132117164,-0.14429930310074,
1.0239876538093));
#22006=CARTESIAN_POINT('Ctrl Pts',(0.445111721969657,-0.0928409665394226,
1.03192403056628));
#22007=CARTESIAN_POINT('Ctrl Pts',(0.440685038163619,-0.0762225747374254,
1.03380912944435));
#22008=CARTESIAN_POINT('Ctrl Pts',(0.437601487681056,-0.05953,1.03511272300331));
#22009=CARTESIAN_POINT('Origin',(0.685838782044607,-0.05953,0.860014630714833));
#22010=CARTESIAN_POINT('Origin',(0.,-0.208355,0.));
#22011=CARTESIAN_POINT('',(0.0548532617164168,-0.05953,1.12247250791415));
#22012=CARTESIAN_POINT('Origin',(0.,-0.05953,0.));
#22013=CARTESIAN_POINT('',(-0.536443649899848,-0.05953,0.987512846410683));
#22014=CARTESIAN_POINT('Ctrl Pts',(0.0548532617164173,-0.0595300000000001,
1.12247250791414));
#22015=CARTESIAN_POINT('Ctrl Pts',(0.05150947068137,-0.0762225747374254,
1.12263591311425));
#22016=CARTESIAN_POINT('Ctrl Pts',(0.0467032526342597,-0.0928409665394227,
1.12285816383385));
#22017=CARTESIAN_POINT('Ctrl Pts',(0.0269302585198975,-0.144299303100741,
1.12357162229597));
#22018=CARTESIAN_POINT('Ctrl Pts',(0.006392292392153,-0.177024326825049,
1.12404235695137));
#22019=CARTESIAN_POINT('Ctrl Pts',(-0.0383992541984087,-0.227269801620063,
1.12335509974011));
#22020=CARTESIAN_POINT('Ctrl Pts',(-0.0680399972366993,-0.251265615809407,
1.12208997038458));
#22021=CARTESIAN_POINT('Ctrl Pts',(-0.117914228755037,-0.279889827963178,
1.1178344036749));
#22022=CARTESIAN_POINT('Ctrl Pts',(-0.14381238480104,-0.290879136862659,
1.11490049012186));
#22023=CARTESIAN_POINT('Ctrl Pts',(-0.19728546073067,-0.305251990234488,
1.10669035995599));
#22024=CARTESIAN_POINT('Ctrl Pts',(-0.224855950742601,-0.308638795020976,
1.10139101611326));
#22025=CARTESIAN_POINT('Ctrl Pts',(-0.275287440920027,-0.308638795020976,
1.0898803575765));
#22026=CARTESIAN_POINT('Ctrl Pts',(-0.302426893214945,-0.305251990234488,
1.08269251410343));
#22027=CARTESIAN_POINT('Ctrl Pts',(-0.35416671187353,-0.290879136862659,
1.06688848765783));
#22028=CARTESIAN_POINT('Ctrl Pts',(-0.3787731215897,-0.279889827963178,
1.05829506364875));
#22029=CARTESIAN_POINT('Ctrl Pts',(-0.425554672694338,-0.251265615809407,
1.04048957871266));
#22030=CARTESIAN_POINT('Ctrl Pts',(-0.452808978448581,-0.227269801620063,
1.02876878445619));
#22031=CARTESIAN_POINT('Ctrl Pts',(-0.493462957200432,-0.177024326825049,
1.0099536580922));
#22032=CARTESIAN_POINT('Ctrl Pts',(-0.511762781179148,-0.14429930310074,
1.00061845128527));
#22033=CARTESIAN_POINT('Ctrl Pts',(-0.529268075276157,-0.0928409665394226,
0.991396466802468));
#22034=CARTESIAN_POINT('Ctrl Pts',(-0.533501897135713,-0.0762225747374254,
0.989110885965947));
#22035=CARTESIAN_POINT('Ctrl Pts',(-0.536443649899848,-0.0595300000000001,
0.987512846410683));
#22036=CARTESIAN_POINT('',(-0.843383895613249,-0.05953,0.742736168477219));
#22037=CARTESIAN_POINT('Origin',(0.,-0.05953,0.));
#22038=CARTESIAN_POINT('',(-1.10653577764992,-0.05953,0.196295654879792));
#22039=CARTESIAN_POINT('Ctrl Pts',(-0.843383895613249,-0.0595300000000001,
0.742736168477219));
#22040=CARTESIAN_POINT('Ctrl Pts',(-0.84559647055299,-0.0762225747374255,
0.740223768851062));
#22041=CARTESIAN_POINT('Ctrl Pts',(-0.848766861100456,-0.0928409665394227,
0.736604687327351));
#22042=CARTESIAN_POINT('Ctrl Pts',(-0.861652925570091,-0.144299303100741,
0.721590372101268));
#22043=CARTESIAN_POINT('Ctrl Pts',(-0.87482617317514,-0.177024326825049,
0.705826641853758));
#22044=CARTESIAN_POINT('Ctrl Pts',(-0.902215926359523,-0.227269801620063,
0.670378702718353));
#22045=CARTESIAN_POINT('Ctrl Pts',(-0.919707509403859,-0.251265615809407,
0.646415841396062));
#22046=CARTESIAN_POINT('Ctrl Pts',(-0.947476448101718,-0.279889827963178,
0.604769294586516));
#22047=CARTESIAN_POINT('Ctrl Pts',(-0.961329858300736,-0.290879136862659,
0.582692035672022));
#22048=CARTESIAN_POINT('Ctrl Pts',(-0.988250837578047,-0.305251990234488,
0.535766169015486));
#22049=CARTESIAN_POINT('Ctrl Pts',(-1.00129756308006,-0.308638795020976,
0.510906605094603));
#22050=CARTESIAN_POINT('Ctrl Pts',(-1.02374168767024,-0.308638795020976,
0.46430090015576));
#22051=CARTESIAN_POINT('Ctrl Pts',(-1.03504317708586,-0.305251990234488,
0.438600874831839));
#22052=CARTESIAN_POINT('Ctrl Pts',(-1.05494634094458,-0.290879136862659,
0.388295406390235));
#22053=CARTESIAN_POINT('Ctrl Pts',(-1.06356957703048,-0.279889827963178,
0.363699428370917));
#22054=CARTESIAN_POINT('Ctrl Pts',(-1.0788165083757,-0.251265615809407,
0.316022600643821));
#22055=CARTESIAN_POINT('Ctrl Pts',(-1.08664560412098,-0.227269801620063,
0.287406530683752));
#22056=CARTESIAN_POINT('Ctrl Pts',(-1.09728268713976,-0.177024326825049,
0.243890930799337));
#22057=CARTESIAN_POINT('Ctrl Pts',(-1.10139388218929,-0.144299303100741,
0.22376314604679));
#22058=CARTESIAN_POINT('Ctrl Pts',(-1.10509821673782,-0.0928409665394227,
0.204327142733961));
#22059=CARTESIAN_POINT('Ctrl Pts',(-1.10595102243643,-0.0762225747374254,
0.199591971170104));
#22060=CARTESIAN_POINT('Ctrl Pts',(-1.10653577764992,-0.0595300000000001,
0.196295654879792));
#22061=CARTESIAN_POINT('',(-1.123812,-0.05953,1.37627276864339E-16));
#22062=CARTESIAN_POINT('Origin',(0.,-0.05953,0.));
#22063=CARTESIAN_POINT('',(-1.123812,-0.35718,1.37627276864339E-16));
#22064=CARTESIAN_POINT('',(-1.123812,-0.208355,1.37627276864339E-16));
#22065=CARTESIAN_POINT('Origin',(0.,-0.35718,0.));
#22066=CARTESIAN_POINT('',(-1.10653577764992,-0.05953,-0.196295654879793));
#22067=CARTESIAN_POINT('Origin',(0.,-0.05953,0.));
#22068=CARTESIAN_POINT('',(-0.843383895613249,-0.05953,-0.742736168477219));
#22069=CARTESIAN_POINT('Ctrl Pts',(-1.10653577764992,-0.0595300000000001,
-0.196295654879792));
#22070=CARTESIAN_POINT('Ctrl Pts',(-1.10595102243643,-0.0762225747374255,
-0.199591971170104));
#22071=CARTESIAN_POINT('Ctrl Pts',(-1.10509821673782,-0.0928409665394228,
-0.204327142733962));
#22072=CARTESIAN_POINT('Ctrl Pts',(-1.10139388218929,-0.144299303100741,
-0.22376314604679));
#22073=CARTESIAN_POINT('Ctrl Pts',(-1.09728268713976,-0.177024326825049,
-0.243890930799338));
#22074=CARTESIAN_POINT('Ctrl Pts',(-1.08664560412098,-0.227269801620063,
-0.287406530683753));
#22075=CARTESIAN_POINT('Ctrl Pts',(-1.0788165083757,-0.251265615809407,
-0.316022600643821));
#22076=CARTESIAN_POINT('Ctrl Pts',(-1.06356957703048,-0.279889827963178,
-0.363699428370918));
#22077=CARTESIAN_POINT('Ctrl Pts',(-1.05494634094458,-0.290879136862659,
-0.388295406390235));
#22078=CARTESIAN_POINT('Ctrl Pts',(-1.03504317708586,-0.305251990234488,
-0.438600874831839));
#22079=CARTESIAN_POINT('Ctrl Pts',(-1.02374168767024,-0.308638795020976,
-0.46430090015576));
#22080=CARTESIAN_POINT('Ctrl Pts',(-1.00129756308006,-0.308638795020976,
-0.510906605094603));
#22081=CARTESIAN_POINT('Ctrl Pts',(-0.988250837578047,-0.305251990234488,
-0.535766169015486));
#22082=CARTESIAN_POINT('Ctrl Pts',(-0.961329858300736,-0.290879136862659,
-0.582692035672022));
#22083=CARTESIAN_POINT('Ctrl Pts',(-0.947476448101718,-0.279889827963178,
-0.604769294586516));
#22084=CARTESIAN_POINT('Ctrl Pts',(-0.919707509403859,-0.251265615809407,
-0.646415841396062));
#22085=CARTESIAN_POINT('Ctrl Pts',(-0.902215926359523,-0.227269801620064,
-0.670378702718353));
#22086=CARTESIAN_POINT('Ctrl Pts',(-0.87482617317514,-0.177024326825049,
-0.705826641853758));
#22087=CARTESIAN_POINT('Ctrl Pts',(-0.861652925570091,-0.144299303100741,
-0.721590372101268));
#22088=CARTESIAN_POINT('Ctrl Pts',(-0.848766861100456,-0.0928409665394229,
-0.736604687327351));
#22089=CARTESIAN_POINT('Ctrl Pts',(-0.84559647055299,-0.0762225747374255,
-0.740223768851063));
#22090=CARTESIAN_POINT('Ctrl Pts',(-0.843383895613249,-0.0595300000000001,
-0.742736168477219));
#22091=CARTESIAN_POINT('',(-0.536443649899847,-0.05953,-0.987512846410683));
#22092=CARTESIAN_POINT('Origin',(0.,-0.05953,0.));
#22093=CARTESIAN_POINT('',(0.0548532617164172,-0.05953,-1.12247250791415));
#22094=CARTESIAN_POINT('Ctrl Pts',(-0.536443649899848,-0.0595300000000001,
-0.987512846410683));
#22095=CARTESIAN_POINT('Ctrl Pts',(-0.533501897135712,-0.0762225747374254,
-0.989110885965947));
#22096=CARTESIAN_POINT('Ctrl Pts',(-0.529268075276156,-0.0928409665394227,
-0.991396466802469));
#22097=CARTESIAN_POINT('Ctrl Pts',(-0.511762781179147,-0.144299303100741,
-1.00061845128527));
#22098=CARTESIAN_POINT('Ctrl Pts',(-0.493462957200432,-0.177024326825049,
-1.0099536580922));
#22099=CARTESIAN_POINT('Ctrl Pts',(-0.45280897844858,-0.227269801620063,
-1.02876878445619));
#22100=CARTESIAN_POINT('Ctrl Pts',(-0.425554672694337,-0.251265615809407,
-1.04048957871266));
#22101=CARTESIAN_POINT('Ctrl Pts',(-0.3787731215897,-0.279889827963178,
-1.05829506364875));
#22102=CARTESIAN_POINT('Ctrl Pts',(-0.354166711873529,-0.290879136862659,
-1.06688848765783));
#22103=CARTESIAN_POINT('Ctrl Pts',(-0.302426893214944,-0.305251990234488,
-1.08269251410343));
#22104=CARTESIAN_POINT('Ctrl Pts',(-0.275287440920027,-0.308638795020976,
-1.0898803575765));
#22105=CARTESIAN_POINT('Ctrl Pts',(-0.224855950742601,-0.308638795020976,
-1.10139101611326));
#22106=CARTESIAN_POINT('Ctrl Pts',(-0.19728546073067,-0.305251990234488,
-1.10669035995599));
#22107=CARTESIAN_POINT('Ctrl Pts',(-0.143812384801039,-0.290879136862659,
-1.11490049012186));
#22108=CARTESIAN_POINT('Ctrl Pts',(-0.117914228755037,-0.279889827963178,
-1.1178344036749));
#22109=CARTESIAN_POINT('Ctrl Pts',(-0.0680399972366989,-0.251265615809407,
-1.12208997038458));
#22110=CARTESIAN_POINT('Ctrl Pts',(-0.0383992541984084,-0.227269801620063,
-1.12335509974011));
#22111=CARTESIAN_POINT('Ctrl Pts',(0.00639229239215326,-0.177024326825049,
-1.12404235695137));
#22112=CARTESIAN_POINT('Ctrl Pts',(0.0269302585198977,-0.144299303100741,
-1.12357162229597));
#22113=CARTESIAN_POINT('Ctrl Pts',(0.04670325263426,-0.0928409665394228,
-1.12285816383385));
#22114=CARTESIAN_POINT('Ctrl Pts',(0.0515094706813703,-0.0762225747374255,
-1.12263591311425));
#22115=CARTESIAN_POINT('Ctrl Pts',(0.0548532617164176,-0.0595300000000001,
-1.12247250791414));
#22116=CARTESIAN_POINT('',(0.437601487681057,-0.05953,-1.03511272300331));
#22117=CARTESIAN_POINT('Origin',(0.,-0.05953,0.));
#22118=CARTESIAN_POINT('',(0.911784794170997,-0.05953,-0.656964154625313));
#22119=CARTESIAN_POINT('Ctrl Pts',(0.437601487681056,-0.0595300000000001,
-1.03511272300331));
#22120=CARTESIAN_POINT('Ctrl Pts',(0.440685038163619,-0.0762225747374255,
-1.03380912944435));
#22121=CARTESIAN_POINT('Ctrl Pts',(0.445111721969657,-0.0928409665394228,
-1.03192403056628));
#22122=CARTESIAN_POINT('Ctrl Pts',(0.463236132117164,-0.144299303100741,
-1.0239876538093));
#22123=CARTESIAN_POINT('Ctrl Pts',(0.481944444320713,-0.177024326825049,
-1.01550068154148));
#22124=CARTESIAN_POINT('Ctrl Pts',(0.522002043615455,-0.227269801620064,
-0.995447160474328));
#22125=CARTESIAN_POINT('Ctrl Pts',(0.548158511259203,-0.251265615809407,
-0.981446681891443));
#22126=CARTESIAN_POINT('Ctrl Pts',(0.591247219971725,-0.279889827963178,
-0.955972930713954));
#22127=CARTESIAN_POINT('Ctrl Pts',(0.613307674922609,-0.290879136862659,
-0.942092777160053));
#22128=CARTESIAN_POINT('Ctrl Pts',(0.657923009631182,-0.305251990234487,
-0.91149460735272));
#22129=CARTESIAN_POINT('Ctrl Pts',(0.680463863683393,-0.308638795020976,
-0.894757676234429));
#22130=CARTESIAN_POINT('Ctrl Pts',(0.720906778729542,-0.308638795020976,
-0.862505527716294));
#22131=CARTESIAN_POINT('Ctrl Pts',(0.742239891936899,-0.305251990234488,
-0.844254137480381));
#22132=CARTESIAN_POINT('Ctrl Pts',(0.781998747691872,-0.290879136862659,
-0.80756613568454));
#22133=CARTESIAN_POINT('Ctrl Pts',(0.800439809856112,-0.279889827963178,
-0.789147407129765));
#22134=CARTESIAN_POINT('Ctrl Pts',(0.834863020612702,-0.251265615809407,
-0.752807465209441));
#22135=CARTESIAN_POINT('Ctrl Pts',(0.854332839576145,-0.227269801620064,
-0.73042219438957));
#22136=CARTESIAN_POINT('Ctrl Pts',(0.882797231409153,-0.177024326825049,
-0.695831250979106));
#22137=CARTESIAN_POINT('Ctrl Pts',(0.895234408667242,-0.144299303100741,
-0.679480524217551));
#22138=CARTESIAN_POINT('Ctrl Pts',(0.907004864562642,-0.0928409665394228,
-0.663576540841106));
#22139=CARTESIAN_POINT('Ctrl Pts',(0.909827729890942,-0.0762225747374256,
-0.659680317203144));
#22140=CARTESIAN_POINT('Ctrl Pts',(0.911784794170998,-0.0595300000000001,
-0.656964154625312));
#22141=CARTESIAN_POINT('',(1.08212377959455,-0.05953,-0.303251606722892));
#22142=CARTESIAN_POINT('Origin',(0.,-0.05953,0.));
#22143=CARTESIAN_POINT('',(1.08212377959455,-0.05953,0.303251606722892));
#22144=CARTESIAN_POINT('Ctrl Pts',(1.08212377959455,-0.0595300000000001,
-0.303251606722892));
#22145=CARTESIAN_POINT('Ctrl Pts',(1.0830271513892,-0.0762225747374255,
-0.300028012588062));
#22146=CARTESIAN_POINT('Ctrl Pts',(1.08431331394788,-0.0928409665394228,
-0.2953917518996));
#22147=CARTESIAN_POINT('Ctrl Pts',(1.08940878963422,-0.144299303100741,
-0.276273267473431));
#22148=CARTESIAN_POINT('Ctrl Pts',(1.09443784939331,-0.177024326825049,
-0.256354979351213));
#22149=CARTESIAN_POINT('Ctrl Pts',(1.10373487993589,-0.227269801620064,
-0.212533521233765));
#22150=CARTESIAN_POINT('Ctrl Pts',(1.10909715583869,-0.251265615809407,
-0.183354415742157));
#22151=CARTESIAN_POINT('Ctrl Pts',(1.1160463456491,-0.279889827963178,-0.133783682657561));
#22152=CARTESIAN_POINT('Ctrl Pts',(1.11894887330541,-0.290879136862659,
-0.107881990270302));
#22153=CARTESIAN_POINT('Ctrl Pts',(1.12284346704144,-0.305251990234488,
-0.0539226701638766));
#22154=CARTESIAN_POINT('Ctrl Pts',(1.123812,-0.308638795020976,-0.025864214957475));
#22155=CARTESIAN_POINT('Ctrl Pts',(1.123812,-0.308638795020976,0.025864214957475));
#22156=CARTESIAN_POINT('Ctrl Pts',(1.12284346704144,-0.305251990234488,
0.0539226701638766));
#22157=CARTESIAN_POINT('Ctrl Pts',(1.11894887330541,-0.290879136862659,
0.107881990270302));
#22158=CARTESIAN_POINT('Ctrl Pts',(1.1160463456491,-0.279889827963178,0.133783682657561));
#22159=CARTESIAN_POINT('Ctrl Pts',(1.10909715583869,-0.251265615809407,
0.183354415742157));
#22160=CARTESIAN_POINT('Ctrl Pts',(1.10373487993589,-0.227269801620064,
0.212533521233765));
#22161=CARTESIAN_POINT('Ctrl Pts',(1.09443784939331,-0.177024326825049,
0.256354979351213));
#22162=CARTESIAN_POINT('Ctrl Pts',(1.08940878963422,-0.144299303100741,
0.276273267473431));
#22163=CARTESIAN_POINT('Ctrl Pts',(1.08431331394788,-0.0928409665394228,
0.2953917518996));
#22164=CARTESIAN_POINT('Ctrl Pts',(1.0830271513892,-0.0762225747374255,
0.300028012588062));
#22165=CARTESIAN_POINT('Ctrl Pts',(1.08212377959455,-0.0595300000000001,
0.303251606722892));
#22166=CARTESIAN_POINT('Origin',(0.,-0.05953,0.));
#22167=CARTESIAN_POINT('Origin',(0.,-0.05953,0.));
#22168=CARTESIAN_POINT('',(0.0589974094846122,-0.05953,1.07456964270265));
#22169=CARTESIAN_POINT('Origin',(0.,-0.05953,0.));
#22170=CARTESIAN_POINT('Origin',(-0.244773027351946,-0.05953,1.07242070340001));
#22171=CARTESIAN_POINT('Origin',(-0.244773027351946,0.,1.07242070340001));
#22172=CARTESIAN_POINT('',(-0.519393123750572,-0.05953,0.942555777842682));
#22173=CARTESIAN_POINT('Ctrl Pts',(-0.519393123750572,-0.05953,0.942555777842682));
#22174=CARTESIAN_POINT('Ctrl Pts',(-0.513714466572041,-0.0925528133349865,
0.945684988399766));
#22175=CARTESIAN_POINT('Ctrl Pts',(-0.503136848051455,-0.124911173756694,
0.951483858396181));
#22176=CARTESIAN_POINT('Ctrl Pts',(-0.47593627990192,-0.177924977804098,
0.965323333309091));
#22177=CARTESIAN_POINT('Ctrl Pts',(-0.460931856495794,-0.199697230012983,
0.972669835243841));
#22178=CARTESIAN_POINT('Ctrl Pts',(-0.426157505475872,-0.237895043532788,
0.988400002689705));
#22179=CARTESIAN_POINT('Ctrl Pts',(-0.406380688682952,-0.254319232363049,
0.996771768218699));
#22180=CARTESIAN_POINT('Ctrl Pts',(-0.364750145543744,-0.28018331644634,
1.01272583306292));
#22181=CARTESIAN_POINT('Ctrl Pts',(-0.340838910881557,-0.29104845371857,
1.02112815447116));
#22182=CARTESIAN_POINT('Ctrl Pts',(-0.290495481564827,-0.30527573347708,
1.036574285215));
#22183=CARTESIAN_POINT('Ctrl Pts',(-0.264056468041074,-0.308638795020976,
1.04359501395068));
#22184=CARTESIAN_POINT('Ctrl Pts',(-0.214892249704082,-0.308638795020976,
1.05481642595959));
#22185=CARTESIAN_POINT('Ctrl Pts',(-0.188025341585962,-0.30527573347708,
1.05996242598502));
#22186=CARTESIAN_POINT('Ctrl Pts',(-0.135965654106109,-0.29104845371857,
1.06788913840721));
#22187=CARTESIAN_POINT('Ctrl Pts',(-0.110776745452494,-0.28018331644634,
1.07069360430242));
#22188=CARTESIAN_POINT('Ctrl Pts',(-0.0663467128214646,-0.254319232363049,
1.07438230428002));
#22189=CARTESIAN_POINT('Ctrl Pts',(-0.0448960436540983,-0.237895043532788,
1.07542044338697));
#22190=CARTESIAN_POINT('Ctrl Pts',(-0.00674037211528124,-0.199697230012983,
1.07633607767727));
#22191=CARTESIAN_POINT('Ctrl Pts',(0.00996567398334777,-0.177924977804098,
1.07622728347683));
#22192=CARTESIAN_POINT('Ctrl Pts',(0.0404772621979741,-0.124911173756694,
1.07556023164702));
#22193=CARTESIAN_POINT('Ctrl Pts',(0.0525234025782719,-0.0925528133349865,
1.07492508698591));
#22194=CARTESIAN_POINT('Ctrl Pts',(0.0589974094846124,-0.05953,1.07456964270265));
#22195=CARTESIAN_POINT('Origin',(-0.244773027351946,-0.05953,1.07242070340001));
#22196=CARTESIAN_POINT('Origin',(0.,-0.05953,0.));
#22197=CARTESIAN_POINT('',(-0.803348093619616,-0.05953,0.716109245731214));
#22198=CARTESIAN_POINT('Origin',(0.,-0.05953,0.));
#22199=CARTESIAN_POINT('Origin',(-0.991065754692661,-0.05953,0.477272113029314));
#22200=CARTESIAN_POINT('Origin',(-0.991065754692661,0.,0.477272113029314));
#22201=CARTESIAN_POINT('',(-1.06075609691358,-0.05953,0.181596019242328));
#22202=CARTESIAN_POINT('Ctrl Pts',(-1.06075609691358,-0.05953,0.181596019242328));
#22203=CARTESIAN_POINT('Ctrl Pts',(-1.05966202740332,-0.0925528133349865,
0.187986803072856));
#22204=CARTESIAN_POINT('Ctrl Pts',(-1.05760072925372,-0.124911173756694,
0.199872254546857));
#22205=CARTESIAN_POINT('Ctrl Pts',(-1.05146158959546,-0.177924977804098,
0.22976728653846));
#22206=CARTESIAN_POINT('Ctrl Pts',(-1.04785021111757,-0.199697230012983,
0.246078686169301));
#22207=CARTESIAN_POINT('Ctrl Pts',(-1.03846709802406,-0.237895043532788,
0.283073967563097));
#22208=CARTESIAN_POINT('Ctrl Pts',(-1.03268176429485,-0.254319232363049,
0.303755815985685));
#22209=CARTESIAN_POINT('Ctrl Pts',(-1.01919893537026,-0.28018331644634,
0.346251081972725));
#22210=CARTESIAN_POINT('Ctrl Pts',(-1.01085972381132,-0.29104845371857,
0.370184399726282));
#22211=CARTESIAN_POINT('Ctrl Pts',(-0.99154738033959,-0.30527573347708,
0.419174982698463));
#22212=CARTESIAN_POINT('Ctrl Pts',(-0.980551951791748,-0.308638795020976,
0.444223188605045));
#22213=CARTESIAN_POINT('Ctrl Pts',(-0.958671816228589,-0.308638795020976,
0.489657758261848));
#22214=CARTESIAN_POINT('Ctrl Pts',(-0.945943877838127,-0.30527573347708,
0.51387163140139));
#22215=CARTESIAN_POINT('Ctrl Pts',(-0.91968254693063,-0.29104845371857,
0.559515758398093));
#22216=CARTESIAN_POINT('Ctrl Pts',(-0.906170138993533,-0.28018331644634,
0.580957796077825));
#22217=CARTESIAN_POINT('Ctrl Pts',(-0.8813524085237,-0.254319232363049,
0.617994461173994));
#22218=CARTESIAN_POINT('Ctrl Pts',(-0.868789784891799,-0.237895043532788,
0.635412538795143));
#22219=CARTESIAN_POINT('Ctrl Pts',(-0.845715984518854,-0.199697230012983,
0.66581473268113));
#22220=CARTESIAN_POINT('Ctrl Pts',(-0.835214876415962,-0.177924977804098,
0.678808213394124));
#22221=CARTESIAN_POINT('Ctrl Pts',(-0.815669690204649,-0.124911173756694,
0.702247233627224));
#22222=CARTESIAN_POINT('Ctrl Pts',(-0.807662468433796,-0.0925528133349865,
0.711269279199861));
#22223=CARTESIAN_POINT('Ctrl Pts',(-0.803348093619616,-0.05953,0.716109245731214));
#22224=CARTESIAN_POINT('Origin',(-0.991065754692661,-0.05953,0.477272113029314));
#22225=CARTESIAN_POINT('Origin',(0.,-0.05953,0.));
#22226=CARTESIAN_POINT('',(-1.076188,-0.05953,1.31795018948079E-16));
#22227=CARTESIAN_POINT('Origin',(0.,-0.05953,0.));
#22228=CARTESIAN_POINT('',(-1.06075609691358,-0.05953,-0.181596019242328));
#22229=CARTESIAN_POINT('Origin',(0.,-0.05953,0.));
#22230=CARTESIAN_POINT('Origin',(-0.991065754692661,-0.05953,-0.477272113029314));
#22231=CARTESIAN_POINT('Origin',(-0.991065754692661,0.,-0.477272113029314));
#22232=CARTESIAN_POINT('',(-0.803348093619616,-0.05953,-0.716109245731215));
#22233=CARTESIAN_POINT('Ctrl Pts',(-0.803348093619616,-0.05953,-0.716109245731215));
#22234=CARTESIAN_POINT('Ctrl Pts',(-0.807662468433795,-0.0925528133349865,
-0.711269279199862));
#22235=CARTESIAN_POINT('Ctrl Pts',(-0.815669690204649,-0.124911173756694,
-0.702247233627224));
#22236=CARTESIAN_POINT('Ctrl Pts',(-0.835214876415962,-0.177924977804098,
-0.678808213394124));
#22237=CARTESIAN_POINT('Ctrl Pts',(-0.845715984518854,-0.199697230012983,
-0.66581473268113));
#22238=CARTESIAN_POINT('Ctrl Pts',(-0.868789784891799,-0.237895043532788,
-0.635412538795143));
#22239=CARTESIAN_POINT('Ctrl Pts',(-0.8813524085237,-0.254319232363049,
-0.617994461173994));
#22240=CARTESIAN_POINT('Ctrl Pts',(-0.906170138993533,-0.28018331644634,
-0.580957796077826));
#22241=CARTESIAN_POINT('Ctrl Pts',(-0.91968254693063,-0.29104845371857,
-0.559515758398093));
#22242=CARTESIAN_POINT('Ctrl Pts',(-0.945943877838127,-0.30527573347708,
-0.51387163140139));
#22243=CARTESIAN_POINT('Ctrl Pts',(-0.958671816228589,-0.308638795020976,
-0.489657758261848));
#22244=CARTESIAN_POINT('Ctrl Pts',(-0.980551951791748,-0.308638795020976,
-0.444223188605045));
#22245=CARTESIAN_POINT('Ctrl Pts',(-0.99154738033959,-0.30527573347708,
-0.419174982698463));
#22246=CARTESIAN_POINT('Ctrl Pts',(-1.01085972381132,-0.29104845371857,
-0.370184399726282));
#22247=CARTESIAN_POINT('Ctrl Pts',(-1.01919893537026,-0.28018331644634,
-0.346251081972725));
#22248=CARTESIAN_POINT('Ctrl Pts',(-1.03268176429485,-0.254319232363049,
-0.303755815985685));
#22249=CARTESIAN_POINT('Ctrl Pts',(-1.03846709802406,-0.237895043532788,
-0.283073967563097));
#22250=CARTESIAN_POINT('Ctrl Pts',(-1.04785021111757,-0.199697230012983,
-0.246078686169302));
#22251=CARTESIAN_POINT('Ctrl Pts',(-1.05146158959546,-0.177924977804098,
-0.229767286538461));
#22252=CARTESIAN_POINT('Ctrl Pts',(-1.05760072925372,-0.124911173756694,
-0.199872254546858));
#22253=CARTESIAN_POINT('Ctrl Pts',(-1.05966202740332,-0.0925528133349864,
-0.187986803072857));
#22254=CARTESIAN_POINT('Ctrl Pts',(-1.06075609691358,-0.05953,-0.181596019242328));
#22255=CARTESIAN_POINT('Origin',(-0.991065754692661,-0.05953,-0.477272113029314));
#22256=CARTESIAN_POINT('Origin',(0.,-0.05953,0.));
#22257=CARTESIAN_POINT('',(-0.519393123750572,-0.05953,-0.942555777842682));
#22258=CARTESIAN_POINT('Origin',(0.,-0.05953,0.));
#22259=CARTESIAN_POINT('Origin',(-0.244773027351946,-0.05953,-1.07242070340001));
#22260=CARTESIAN_POINT('Origin',(-0.244773027351946,0.,-1.07242070340001));
#22261=CARTESIAN_POINT('',(0.0589974094846125,-0.05953,-1.07456964270265));
#22262=CARTESIAN_POINT('Ctrl Pts',(0.0589974094846127,-0.05953,-1.07456964270265));
#22263=CARTESIAN_POINT('Ctrl Pts',(0.0525234025782722,-0.0925528133349865,
-1.07492508698591));
#22264=CARTESIAN_POINT('Ctrl Pts',(0.0404772621979744,-0.124911173756694,
-1.07556023164702));
#22265=CARTESIAN_POINT('Ctrl Pts',(0.0099656739833481,-0.177924977804098,
-1.07622728347683));
#22266=CARTESIAN_POINT('Ctrl Pts',(-0.00674037211528096,-0.199697230012983,
-1.07633607767727));
#22267=CARTESIAN_POINT('Ctrl Pts',(-0.044896043654098,-0.237895043532788,
-1.07542044338697));
#22268=CARTESIAN_POINT('Ctrl Pts',(-0.0663467128214644,-0.254319232363049,
-1.07438230428002));
#22269=CARTESIAN_POINT('Ctrl Pts',(-0.110776745452493,-0.28018331644634,
-1.07069360430242));
#22270=CARTESIAN_POINT('Ctrl Pts',(-0.135965654106109,-0.29104845371857,
-1.06788913840721));
#22271=CARTESIAN_POINT('Ctrl Pts',(-0.188025341585962,-0.30527573347708,
-1.05996242598502));
#22272=CARTESIAN_POINT('Ctrl Pts',(-0.214892249704082,-0.308638795020976,
-1.05481642595959));
#22273=CARTESIAN_POINT('Ctrl Pts',(-0.264056468041074,-0.308638795020976,
-1.04359501395068));
#22274=CARTESIAN_POINT('Ctrl Pts',(-0.290495481564827,-0.30527573347708,
-1.036574285215));
#22275=CARTESIAN_POINT('Ctrl Pts',(-0.340838910881557,-0.291048453718569,
-1.02112815447116));
#22276=CARTESIAN_POINT('Ctrl Pts',(-0.364750145543744,-0.28018331644634,
-1.01272583306292));
#22277=CARTESIAN_POINT('Ctrl Pts',(-0.406380688682952,-0.254319232363049,
-0.996771768218699));
#22278=CARTESIAN_POINT('Ctrl Pts',(-0.426157505475872,-0.237895043532788,
-0.988400002689705));
#22279=CARTESIAN_POINT('Ctrl Pts',(-0.460931856495794,-0.199697230012983,
-0.972669835243841));
#22280=CARTESIAN_POINT('Ctrl Pts',(-0.475936279901919,-0.177924977804098,
-0.965323333309091));
#22281=CARTESIAN_POINT('Ctrl Pts',(-0.503136848051454,-0.124911173756694,
-0.951483858396181));
#22282=CARTESIAN_POINT('Ctrl Pts',(-0.513714466572041,-0.0925528133349865,
-0.945684988399766));
#22283=CARTESIAN_POINT('Ctrl Pts',(-0.519393123750572,-0.05953,-0.942555777842682));
#22284=CARTESIAN_POINT('Origin',(-0.244773027351946,-0.05953,-1.07242070340001));
#22285=CARTESIAN_POINT('Origin',(0.,-0.05953,0.));
#22286=CARTESIAN_POINT('',(0.413083465285518,-0.05953,-0.993751811093549));
#22287=CARTESIAN_POINT('Origin',(0.,-0.05953,0.));
#22288=CARTESIAN_POINT('Origin',(0.685838782044607,-0.05953,-0.860014630714833));
#22289=CARTESIAN_POINT('Origin',(0.685838782044607,0.,-0.860014630714833));
#22290=CARTESIAN_POINT('',(0.876916659919095,-0.05953,-0.623857181492959));
#22291=CARTESIAN_POINT('Ctrl Pts',(0.876916659919095,-0.05953,-0.623857181492958));
#22292=CARTESIAN_POINT('Ctrl Pts',(0.873158080166742,-0.0925528133349865,
-0.62914037979579));
#22293=CARTESIAN_POINT('Ctrl Pts',(0.866144010579847,-0.124911173756694,
-0.638954437806245));
#22294=CARTESIAN_POINT('Ctrl Pts',(0.847641868610495,-0.177924977804098,
-0.663225258065736));
#22295=CARTESIAN_POINT('Ctrl Pts',(0.837310877969633,-0.199697230012983,
-0.676354402927683));
#22296=CARTESIAN_POINT('Ctrl Pts',(0.81280533416753,-0.237895043532788,
-0.705614819529209));
#22297=CARTESIAN_POINT('Ctrl Pts',(0.798619410861634,-0.254319232363049,
-0.721738358858166));
#22298=CARTESIAN_POINT('Ctrl Pts',(0.768033796848072,-0.28018331644634,
-0.754175290318038));
#22299=CARTESIAN_POINT('Ctrl Pts',(0.750136149454208,-0.29104845371857,
-0.772120216227122));
#22300=CARTESIAN_POINT('Ctrl Pts',(0.711480111898423,-0.30527573347708,
-0.807879894508811));
#22301=CARTESIAN_POINT('Ctrl Pts',(0.690705563850638,-0.308638795020976,
-0.825676810575913));
#22302=CARTESIAN_POINT('Ctrl Pts',(0.651278921914856,-0.308638795020976,
-0.857118508332695));
#22303=CARTESIAN_POINT('Ctrl Pts',(0.629305439856167,-0.30527573347708,
-0.873412008702649));
#22304=CARTESIAN_POINT('Ctrl Pts',(0.585840553788742,-0.29104845371857,
-0.903141581680914));
#22305=CARTESIAN_POINT('Ctrl Pts',(0.564362943424239,-0.28018331644634,
-0.916597376014514));
#22306=CARTESIAN_POINT('Ctrl Pts',(0.525933334162556,-0.254319232363049,
-0.939198248544427));
#22307=CARTESIAN_POINT('Ctrl Pts',(0.507057380724533,-0.237895043532788,
-0.949440676105255));
#22308=CARTESIAN_POINT('Ctrl Pts',(0.473077587363686,-0.199697230012983,
-0.966820759530997));
#22309=CARTESIAN_POINT('Ctrl Pts',(0.457978755888596,-0.177924977804098,
-0.973971221090534));
#22310=CARTESIAN_POINT('Ctrl Pts',(0.430199341854858,-0.124911173756694,
-0.986608710139579));
#22311=CARTESIAN_POINT('Ctrl Pts',(0.419070565453384,-0.0925528133349865,
-0.991263089003441));
#22312=CARTESIAN_POINT('Ctrl Pts',(0.413083465285518,-0.05953,-0.993751811093549));
#22313=CARTESIAN_POINT('Origin',(0.685838782044607,-0.05953,-0.860014630714833));
#22314=CARTESIAN_POINT('Origin',(0.,-0.208355,0.));
#22315=CARTESIAN_POINT('',(-1.076188,-0.35718,1.31795018948079E-16));
#22316=CARTESIAN_POINT('Origin',(0.,-0.35718,0.));
#22317=CARTESIAN_POINT('',(-1.076188,-0.208355,1.31795018948079E-16));
#22318=CARTESIAN_POINT('',(1.03449977959455,-0.05953,0.296632461748266));
#22319=CARTESIAN_POINT('Origin',(0.,-0.05953,0.));
#22320=CARTESIAN_POINT('',(1.03449977959455,-0.05953,-0.296632461748266));
#22321=CARTESIAN_POINT('Ctrl Pts',(1.03449977959455,-0.05953,0.296632461748267));
#22322=CARTESIAN_POINT('Ctrl Pts',(1.03628691421076,-0.0925528133349865,
0.290399865505497));
#22323=CARTESIAN_POINT('Ctrl Pts',(1.03958665287714,-0.124911173756694,
0.278797079997872));
#22324=CARTESIAN_POINT('Ctrl Pts',(1.0470264474309,-0.177924977804098,0.249198913998601));
#22325=CARTESIAN_POINT('Ctrl Pts',(1.05084995891418,-0.199697230012983,
0.232935932341942));
#22326=CARTESIAN_POINT('Ctrl Pts',(1.05844771715377,-0.237895043532788,
0.195533155353269));
#22327=CARTESIAN_POINT('Ctrl Pts',(1.06220882929878,-0.254319232363049,
0.17438929156337));
#22328=CARTESIAN_POINT('Ctrl Pts',(1.06849922508772,-0.28018331644634,0.130252399648131));
#22329=CARTESIAN_POINT('Ctrl Pts',(1.07137013248666,-0.29104845371857,0.105070977154072));
#22330=CARTESIAN_POINT('Ctrl Pts',(1.07522652957392,-0.30527573347708,0.0525526752791107));
#22331=CARTESIAN_POINT('Ctrl Pts',(1.076188,-0.308638795020976,0.025214283908933));
#22332=CARTESIAN_POINT('Ctrl Pts',(1.076188,-0.308638795020976,-0.025214283908933));
#22333=CARTESIAN_POINT('Ctrl Pts',(1.07522652957392,-0.30527573347708,-0.0525526752791107));
#22334=CARTESIAN_POINT('Ctrl Pts',(1.07137013248666,-0.29104845371857,-0.105070977154072));
#22335=CARTESIAN_POINT('Ctrl Pts',(1.06849922508772,-0.28018331644634,-0.130252399648131));
#22336=CARTESIAN_POINT('Ctrl Pts',(1.06220882929878,-0.254319232363049,
-0.17438929156337));
#22337=CARTESIAN_POINT('Ctrl Pts',(1.05844771715377,-0.237895043532788,
-0.195533155353269));
#22338=CARTESIAN_POINT('Ctrl Pts',(1.05084995891418,-0.199697230012983,
-0.232935932341942));
#22339=CARTESIAN_POINT('Ctrl Pts',(1.0470264474309,-0.177924977804098,-0.249198913998601));
#22340=CARTESIAN_POINT('Ctrl Pts',(1.03958665287714,-0.124911173756694,
-0.278797079997872));
#22341=CARTESIAN_POINT('Ctrl Pts',(1.03628691421076,-0.0925528133349865,
-0.290399865505497));
#22342=CARTESIAN_POINT('Ctrl Pts',(1.03449977959455,-0.05953,-0.296632461748267));
#22343=CARTESIAN_POINT('Origin',(0.,-0.05953,0.));
#22344=CARTESIAN_POINT('Origin',(0.,-0.05953,0.));
#22345=CARTESIAN_POINT('Origin',(1.1,-0.05953,0.));
#22346=CARTESIAN_POINT('Origin',(1.1,0.,0.));
#22347=CARTESIAN_POINT('Origin',(1.1,-0.05953,0.));
#22348=CARTESIAN_POINT('Origin',(0.,-0.35718,0.));
#22349=CARTESIAN_POINT('Origin',(0.,-0.05953,0.));
#23575=UNCERTAINTY_MEASURE_WITH_UNIT(LENGTH_MEASURE(0.001),#23729,
'DISTANCE_ACCURACY_VALUE',
'Maximum model space distance between geometric entities at asserted c
onnectivities');
#23611=UNCERTAINTY_MEASURE_WITH_UNIT(LENGTH_MEASURE(0.001),#23729,
'DISTANCE_ACCURACY_VALUE',
'Maximum model space distance between geometric entities at asserted c
onnectivities');
#23692=(
GEOMETRIC_REPRESENTATION_CONTEXT(3)
GLOBAL_UNCERTAINTY_ASSIGNED_CONTEXT((#23575))
GLOBAL_UNIT_ASSIGNED_CONTEXT((#23729,#23731,#23732))
REPRESENTATION_CONTEXT('','3D')
);
#23728=(
GEOMETRIC_REPRESENTATION_CONTEXT(3)
GLOBAL_UNCERTAINTY_ASSIGNED_CONTEXT((#23611))
GLOBAL_UNIT_ASSIGNED_CONTEXT((#23729,#23731,#23732))
REPRESENTATION_CONTEXT('','3D')
);
#23729=(
LENGTH_UNIT()
NAMED_UNIT(*)
SI_UNIT(.CENTI.,.METRE.)
);
#23731=(
NAMED_UNIT(*)
PLANE_ANGLE_UNIT()
SI_UNIT($,.RADIAN.)
);
#23732=(
NAMED_UNIT(*)
SI_UNIT($,.STERADIAN.)
SOLID_ANGLE_UNIT()
);
#23813=SHAPE_DEFINITION_REPRESENTATION(#23929,#24192);
#23929=PRODUCT_DEFINITION_SHAPE('',$,#24309);
#24192=SHAPE_REPRESENTATION('',(#14829),#23692);
#24228=PRODUCT_DEFINITION_CONTEXT('part definition',#24578,'design');
#24309=PRODUCT_DEFINITION('Cage','Cage',#24425,#24228);
#24425=PRODUCT_DEFINITION_FORMATION('',$,#24660);
#24578=APPLICATION_CONTEXT(
'Core Data for Automotive Mechanical Design Process');
#24579=PRODUCT_CONTEXT('part definition',#24578,'mechanical');
#24660=PRODUCT('Cage','Cage','Cage',(#24579));
#24759=COLOUR_RGB('Grey',0.48,0.52,0.57);
#24760=FILL_AREA_STYLE_COLOUR('',#24759);
#24761=FILL_AREA_STYLE('',(#24760));
#24762=SURFACE_STYLE_FILL_AREA(#24761);
#24763=SURFACE_SIDE_STYLE('',(#24762));
#24764=SURFACE_STYLE_USAGE(.BOTH.,#24763);
#24765=PRESENTATION_STYLE_ASSIGNMENT((#24764));
ENDSEC;
END-ISO-10303-21;
